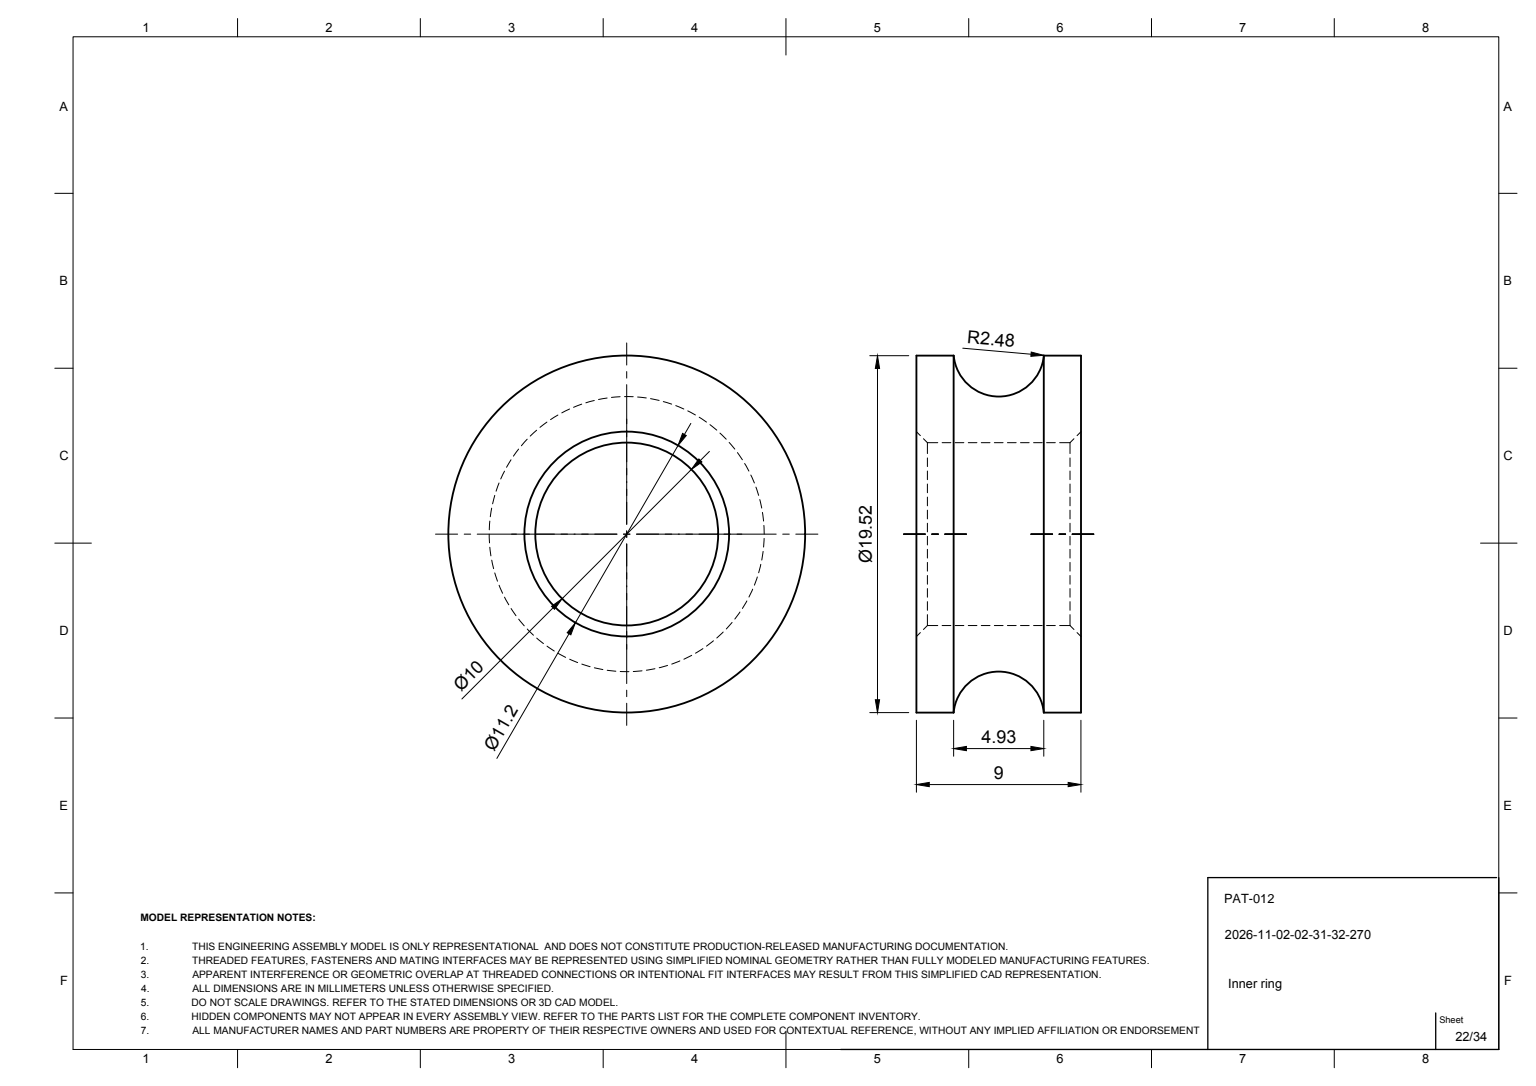
ISO-10303-21;
HEADER;
/* Generated by software containing ST-Developer
 * from STEP Tools, Inc. (www.steptools.com) 
 */

FILE_DESCRIPTION(
/* description */ ('Belt tensioner idler arm'),
/* implementation_level */ '2;1');

FILE_NAME(
/* name */ 'Inner ring.step',
/* time_stamp */ '2026-10-28T03:22:15-07:00',
/* author */ (''),
/* organization */ (''),
/* preprocessor_version */ 'ST-DEVELOPER v20.2',
/* originating_system */ 'Autodesk Translation Framework v15.17.0.0',
/* authorisation */ '');

FILE_SCHEMA (('AUTOMOTIVE_DESIGN { 1 0 10303 214 3 1 1 }'));
ENDSEC;

DATA;
#10=MECHANICAL_DESIGN_GEOMETRIC_PRESENTATION_REPRESENTATION('',(#465),#12779);
#271=TOROIDAL_SURFACE('',#6968,1.,0.247676);
#304=CONICAL_SURFACE('',#6979,0.53,0.785398163397448);
#305=CONICAL_SURFACE('',#6986,0.53,0.785398163397448);
#397=SHAPE_REPRESENTATION_RELATIONSHIP('SRR','None',#12945,#431);
#431=ADVANCED_BREP_SHAPE_REPRESENTATION('',(#505),#12762);
#465=STYLED_ITEM('',(#13184),#505);
#505=MANIFOLD_SOLID_BREP('Body1',#6201);
#627=FACE_BOUND('',#1495,.T.);
#628=FACE_BOUND('',#1498,.T.);
#765=PLANE('',#6981);
#766=PLANE('',#6984);
#1023=FACE_OUTER_BOUND('',#1490,.T.);
#1024=FACE_OUTER_BOUND('',#1491,.T.);
#1025=FACE_OUTER_BOUND('',#1492,.T.);
#1026=FACE_OUTER_BOUND('',#1493,.T.);
#1027=FACE_OUTER_BOUND('',#1494,.T.);
#1028=FACE_OUTER_BOUND('',#1496,.T.);
#1029=FACE_OUTER_BOUND('',#1497,.T.);
#1030=FACE_OUTER_BOUND('',#1499,.T.);
#1490=EDGE_LOOP('',(#4860,#4861,#4862,#4863,#4864,#4865));
#1491=EDGE_LOOP('',(#4866,#4867,#4868,#4869,#4870));
#1492=EDGE_LOOP('',(#4871,#4872,#4873,#4874));
#1493=EDGE_LOOP('',(#4875,#4876,#4877,#4878));
#1494=EDGE_LOOP('',(#4879));
#1495=EDGE_LOOP('',(#4880));
#1496=EDGE_LOOP('',(#4881,#4882,#4883,#4884,#4885));
#1497=EDGE_LOOP('',(#4886));
#1498=EDGE_LOOP('',(#4887));
#1499=EDGE_LOOP('',(#4888,#4889,#4890,#4891));
#1907=LINE('',#11098,#2256);
#1908=LINE('',#11104,#2257);
#1909=LINE('',#11108,#2258);
#1910=LINE('',#11114,#2259);
#1911=LINE('',#11119,#2260);
#2256=VECTOR('',#8379,0.976185);
#2257=VECTOR('',#8386,0.5);
#2258=VECTOR('',#8391,0.53);
#2259=VECTOR('',#8400,0.976185);
#2260=VECTOR('',#8407,0.53);
#2562=CIRCLE('',#6969,0.976185);
#2563=CIRCLE('',#6970,0.976185);
#2564=CIRCLE('',#6971,0.247676);
#2565=CIRCLE('',#6972,0.976185);
#2566=CIRCLE('',#6973,0.976185);
#2567=CIRCLE('',#6975,0.976185);
#2568=CIRCLE('',#6977,0.5);
#2569=CIRCLE('',#6978,0.5);
#2570=CIRCLE('',#6980,0.56);
#2571=CIRCLE('',#6983,0.976185);
#2572=CIRCLE('',#6985,0.56);
#3020=VERTEX_POINT('',#11087);
#3021=VERTEX_POINT('',#11088);
#3022=VERTEX_POINT('',#11091);
#3023=VERTEX_POINT('',#11093);
#3024=VERTEX_POINT('',#11097);
#3025=VERTEX_POINT('',#11101);
#3026=VERTEX_POINT('',#11103);
#3027=VERTEX_POINT('',#11107);
#3028=VERTEX_POINT('',#11112);
#3029=VERTEX_POINT('',#11116);
#3685=EDGE_CURVE('',#3020,#3021,#2562,.T.);
#3686=EDGE_CURVE('',#3021,#3020,#2563,.T.);
#3687=EDGE_CURVE('',#3021,#3022,#2564,.T.);
#3688=EDGE_CURVE('',#3023,#3022,#2565,.T.);
#3689=EDGE_CURVE('',#3022,#3023,#2566,.T.);
#3690=EDGE_CURVE('',#3023,#3024,#1907,.T.);
#3691=EDGE_CURVE('',#3024,#3024,#2567,.T.);
#3692=EDGE_CURVE('',#3025,#3025,#2568,.T.);
#3693=EDGE_CURVE('',#3025,#3026,#1908,.T.);
#3694=EDGE_CURVE('',#3026,#3026,#2569,.T.);
#3695=EDGE_CURVE('',#3026,#3027,#1909,.T.);
#3696=EDGE_CURVE('',#3027,#3027,#2570,.T.);
#3697=EDGE_CURVE('',#3028,#3028,#2571,.T.);
#3698=EDGE_CURVE('',#3028,#3020,#1910,.T.);
#3699=EDGE_CURVE('',#3029,#3029,#2572,.T.);
#3700=EDGE_CURVE('',#3029,#3025,#1911,.T.);
#4860=ORIENTED_EDGE('',*,*,#3685,.F.);
#4861=ORIENTED_EDGE('',*,*,#3686,.F.);
#4862=ORIENTED_EDGE('',*,*,#3687,.T.);
#4863=ORIENTED_EDGE('',*,*,#3688,.F.);
#4864=ORIENTED_EDGE('',*,*,#3689,.F.);
#4865=ORIENTED_EDGE('',*,*,#3687,.F.);
#4866=ORIENTED_EDGE('',*,*,#3688,.T.);
#4867=ORIENTED_EDGE('',*,*,#3689,.T.);
#4868=ORIENTED_EDGE('',*,*,#3690,.T.);
#4869=ORIENTED_EDGE('',*,*,#3691,.T.);
#4870=ORIENTED_EDGE('',*,*,#3690,.F.);
#4871=ORIENTED_EDGE('',*,*,#3692,.T.);
#4872=ORIENTED_EDGE('',*,*,#3693,.T.);
#4873=ORIENTED_EDGE('',*,*,#3694,.F.);
#4874=ORIENTED_EDGE('',*,*,#3693,.F.);
#4875=ORIENTED_EDGE('',*,*,#3694,.T.);
#4876=ORIENTED_EDGE('',*,*,#3695,.T.);
#4877=ORIENTED_EDGE('',*,*,#3696,.F.);
#4878=ORIENTED_EDGE('',*,*,#3695,.F.);
#4879=ORIENTED_EDGE('',*,*,#3691,.F.);
#4880=ORIENTED_EDGE('',*,*,#3696,.T.);
#4881=ORIENTED_EDGE('',*,*,#3697,.F.);
#4882=ORIENTED_EDGE('',*,*,#3698,.T.);
#4883=ORIENTED_EDGE('',*,*,#3685,.T.);
#4884=ORIENTED_EDGE('',*,*,#3686,.T.);
#4885=ORIENTED_EDGE('',*,*,#3698,.F.);
#4886=ORIENTED_EDGE('',*,*,#3697,.T.);
#4887=ORIENTED_EDGE('',*,*,#3699,.F.);
#4888=ORIENTED_EDGE('',*,*,#3699,.T.);
#4889=ORIENTED_EDGE('',*,*,#3700,.T.);
#4890=ORIENTED_EDGE('',*,*,#3692,.F.);
#4891=ORIENTED_EDGE('',*,*,#3700,.F.);
#5734=CYLINDRICAL_SURFACE('',#6974,0.976185);
#5735=CYLINDRICAL_SURFACE('',#6976,0.5);
#5736=CYLINDRICAL_SURFACE('',#6982,0.976185);
#6000=ADVANCED_FACE('',(#1023),#271,.F.);
#6001=ADVANCED_FACE('',(#1024),#5734,.T.);
#6002=ADVANCED_FACE('',(#1025),#5735,.F.);
#6003=ADVANCED_FACE('',(#1026),#304,.F.);
#6004=ADVANCED_FACE('',(#1027,#627),#765,.T.);
#6005=ADVANCED_FACE('',(#1028),#5736,.T.);
#6006=ADVANCED_FACE('',(#1029,#628),#766,.T.);
#6007=ADVANCED_FACE('',(#1030),#305,.F.);
#6201=CLOSED_SHELL('',(#6000,#6001,#6002,#6003,#6004,#6005,#6006,#6007));
#6967=AXIS2_PLACEMENT_3D('',#11085,#8363,#8364);
#6968=AXIS2_PLACEMENT_3D('',#11086,#8365,#8366);
#6969=AXIS2_PLACEMENT_3D('',#11089,#8367,#8368);
#6970=AXIS2_PLACEMENT_3D('',#11090,#8369,#8370);
#6971=AXIS2_PLACEMENT_3D('',#11092,#8371,#8372);
#6972=AXIS2_PLACEMENT_3D('',#11094,#8373,#8374);
#6973=AXIS2_PLACEMENT_3D('',#11095,#8375,#8376);
#6974=AXIS2_PLACEMENT_3D('',#11096,#8377,#8378);
#6975=AXIS2_PLACEMENT_3D('',#11099,#8380,#8381);
#6976=AXIS2_PLACEMENT_3D('',#11100,#8382,#8383);
#6977=AXIS2_PLACEMENT_3D('',#11102,#8384,#8385);
#6978=AXIS2_PLACEMENT_3D('',#11105,#8387,#8388);
#6979=AXIS2_PLACEMENT_3D('',#11106,#8389,#8390);
#6980=AXIS2_PLACEMENT_3D('',#11109,#8392,#8393);
#6981=AXIS2_PLACEMENT_3D('',#11110,#8394,#8395);
#6982=AXIS2_PLACEMENT_3D('',#11111,#8396,#8397);
#6983=AXIS2_PLACEMENT_3D('',#11113,#8398,#8399);
#6984=AXIS2_PLACEMENT_3D('',#11115,#8401,#8402);
#6985=AXIS2_PLACEMENT_3D('',#11117,#8403,#8404);
#6986=AXIS2_PLACEMENT_3D('',#11118,#8405,#8406);
#8363=DIRECTION('axis',(0.,0.,1.));
#8364=DIRECTION('refdir',(1.,0.,0.));
#8365=DIRECTION('center_axis',(0.,-1.,0.));
#8366=DIRECTION('ref_axis',(0.,0.,-1.));
#8367=DIRECTION('center_axis',(0.,-1.,0.));
#8368=DIRECTION('ref_axis',(1.,0.,0.));
#8369=DIRECTION('center_axis',(0.,-1.,0.));
#8370=DIRECTION('ref_axis',(1.,0.,0.));
#8371=DIRECTION('center_axis',(1.,0.,1.22464679914735E-16));
#8372=DIRECTION('ref_axis',(-1.22464679914735E-16,0.,1.));
#8373=DIRECTION('center_axis',(0.,1.,0.));
#8374=DIRECTION('ref_axis',(1.,0.,0.));
#8375=DIRECTION('center_axis',(0.,1.,0.));
#8376=DIRECTION('ref_axis',(1.,0.,0.));
#8377=DIRECTION('center_axis',(0.,-1.,0.));
#8378=DIRECTION('ref_axis',(1.,0.,0.));
#8379=DIRECTION('',(0.,1.,0.));
#8380=DIRECTION('center_axis',(0.,-1.,0.));
#8381=DIRECTION('ref_axis',(1.,0.,0.));
#8382=DIRECTION('center_axis',(0.,-1.,0.));
#8383=DIRECTION('ref_axis',(1.,0.,0.));
#8384=DIRECTION('center_axis',(0.,-1.,0.));
#8385=DIRECTION('ref_axis',(1.,0.,0.));
#8386=DIRECTION('',(0.,1.,0.));
#8387=DIRECTION('center_axis',(0.,-1.,0.));
#8388=DIRECTION('ref_axis',(1.,0.,0.));
#8389=DIRECTION('center_axis',(0.,1.,0.));
#8390=DIRECTION('ref_axis',(1.,0.,0.));
#8391=DIRECTION('',(-0.707106781186547,0.707106781186548,-8.65956056235493E-17));
#8392=DIRECTION('center_axis',(0.,-1.,0.));
#8393=DIRECTION('ref_axis',(1.,0.,0.));
#8394=DIRECTION('center_axis',(0.,1.,0.));
#8395=DIRECTION('ref_axis',(0.,0.,1.));
#8396=DIRECTION('center_axis',(0.,-1.,0.));
#8397=DIRECTION('ref_axis',(1.,0.,0.));
#8398=DIRECTION('center_axis',(0.,-1.,0.));
#8399=DIRECTION('ref_axis',(1.,0.,0.));
#8400=DIRECTION('',(0.,1.,0.));
#8401=DIRECTION('center_axis',(0.,-1.,0.));
#8402=DIRECTION('ref_axis',(0.,0.,-1.));
#8403=DIRECTION('center_axis',(0.,-1.,0.));
#8404=DIRECTION('ref_axis',(1.,0.,0.));
#8405=DIRECTION('center_axis',(0.,-1.,0.));
#8406=DIRECTION('ref_axis',(1.,0.,0.));
#8407=DIRECTION('',(0.707106781186547,0.707106781186548,8.65956056235493E-17));
#11085=CARTESIAN_POINT('',(0.,0.,0.));
#11086=CARTESIAN_POINT('Origin',(0.,0.,0.));
#11087=CARTESIAN_POINT('',(-0.976185,-0.246528389340863,-1.19548183562566E-16));
#11088=CARTESIAN_POINT('',(-1.19548183562566E-16,-0.246528389340863,0.976185));
#11089=CARTESIAN_POINT('Origin',(0.,-0.246528389340863,0.));
#11090=CARTESIAN_POINT('Origin',(0.,-0.246528389340863,0.));
#11091=CARTESIAN_POINT('',(-1.19548183562566E-16,0.246528389340863,0.976185));
#11092=CARTESIAN_POINT('Origin',(-1.22464679914735E-16,0.,1.));
#11093=CARTESIAN_POINT('',(-0.976185,0.246528389340863,1.19548183562566E-16));
#11094=CARTESIAN_POINT('Origin',(0.,0.246528389340863,0.));
#11095=CARTESIAN_POINT('Origin',(0.,0.246528389340863,0.));
#11096=CARTESIAN_POINT('Origin',(0.,0.,0.));
#11097=CARTESIAN_POINT('',(-0.976185,0.45,-1.19548183562566E-16));
#11098=CARTESIAN_POINT('',(-0.976185,0.,-1.19548183562566E-16));
#11099=CARTESIAN_POINT('Origin',(0.,0.45,0.));
#11100=CARTESIAN_POINT('Origin',(0.,0.,0.));
#11101=CARTESIAN_POINT('',(-0.5,-0.39,-6.12323399573677E-17));
#11102=CARTESIAN_POINT('Origin',(0.,-0.39,0.));
#11103=CARTESIAN_POINT('',(-0.5,0.39,-6.12323399573677E-17));
#11104=CARTESIAN_POINT('',(-0.5,0.,-6.12323399573677E-17));
#11105=CARTESIAN_POINT('Origin',(0.,0.39,0.));
#11106=CARTESIAN_POINT('Origin',(0.,0.42,0.));
#11107=CARTESIAN_POINT('',(-0.56,0.45,-6.85802207522518E-17));
#11108=CARTESIAN_POINT('',(-0.53,0.42,-6.49062803548097E-17));
#11109=CARTESIAN_POINT('Origin',(0.,0.45,0.));
#11110=CARTESIAN_POINT('Origin',(0.976185,0.45,0.));
#11111=CARTESIAN_POINT('Origin',(0.,0.,0.));
#11112=CARTESIAN_POINT('',(-0.976185,-0.45,-1.19548183562566E-16));
#11113=CARTESIAN_POINT('Origin',(0.,-0.45,0.));
#11114=CARTESIAN_POINT('',(-0.976185,0.,-1.19548183562566E-16));
#11115=CARTESIAN_POINT('Origin',(0.56,-0.45,0.));
#11116=CARTESIAN_POINT('',(-0.56,-0.45,-6.85802207522518E-17));
#11117=CARTESIAN_POINT('Origin',(0.,-0.45,0.));
#11118=CARTESIAN_POINT('Origin',(0.,-0.42,0.));
#11119=CARTESIAN_POINT('',(-0.53,-0.42,-6.49062803548097E-17));
#12722=UNCERTAINTY_MEASURE_WITH_UNIT(LENGTH_MEASURE(0.001),#12780,
'DISTANCE_ACCURACY_VALUE',
'Maximum model space distance between geometric entities at asserted c
onnectivities');
#12739=UNCERTAINTY_MEASURE_WITH_UNIT(LENGTH_MEASURE(0.001),#12780,
'DISTANCE_ACCURACY_VALUE',
'Maximum model space distance between geometric entities at asserted c
onnectivities');
#12762=(
GEOMETRIC_REPRESENTATION_CONTEXT(3)
GLOBAL_UNCERTAINTY_ASSIGNED_CONTEXT((#12722))
GLOBAL_UNIT_ASSIGNED_CONTEXT((#12780,#12782,#12783))
REPRESENTATION_CONTEXT('','3D')
);
#12779=(
GEOMETRIC_REPRESENTATION_CONTEXT(3)
GLOBAL_UNCERTAINTY_ASSIGNED_CONTEXT((#12739))
GLOBAL_UNIT_ASSIGNED_CONTEXT((#12780,#12782,#12783))
REPRESENTATION_CONTEXT('','3D')
);
#12780=(
LENGTH_UNIT()
NAMED_UNIT(*)
SI_UNIT(.CENTI.,.METRE.)
);
#12782=(
NAMED_UNIT(*)
PLANE_ANGLE_UNIT()
SI_UNIT($,.RADIAN.)
);
#12783=(
NAMED_UNIT(*)
SI_UNIT($,.STERADIAN.)
SOLID_ANGLE_UNIT()
);
#12806=SHAPE_DEFINITION_REPRESENTATION(#12845,#12945);
#12845=PRODUCT_DEFINITION_SHAPE('',$,#12985);
#12945=SHAPE_REPRESENTATION('',(#6967),#12762);
#12962=PRODUCT_DEFINITION_CONTEXT('part definition',#13081,'design');
#12985=PRODUCT_DEFINITION('Inner ring','Inner ring',#13024,#12962);
#13024=PRODUCT_DEFINITION_FORMATION('',$,#13105);
#13081=APPLICATION_CONTEXT(
'Core Data for Automotive Mechanical Design Process');
#13082=PRODUCT_CONTEXT('part definition',#13081,'mechanical');
#13105=PRODUCT('Inner ring','Inner ring','Inner ring',(#13082));
#13178=COLOUR_RGB('Grey',0.48,0.52,0.57);
#13179=FILL_AREA_STYLE_COLOUR('',#13178);
#13180=FILL_AREA_STYLE('',(#13179));
#13181=SURFACE_STYLE_FILL_AREA(#13180);
#13182=SURFACE_SIDE_STYLE('',(#13181));
#13183=SURFACE_STYLE_USAGE(.BOTH.,#13182);
#13184=PRESENTATION_STYLE_ASSIGNMENT((#13183));
ENDSEC;
END-ISO-10303-21;
